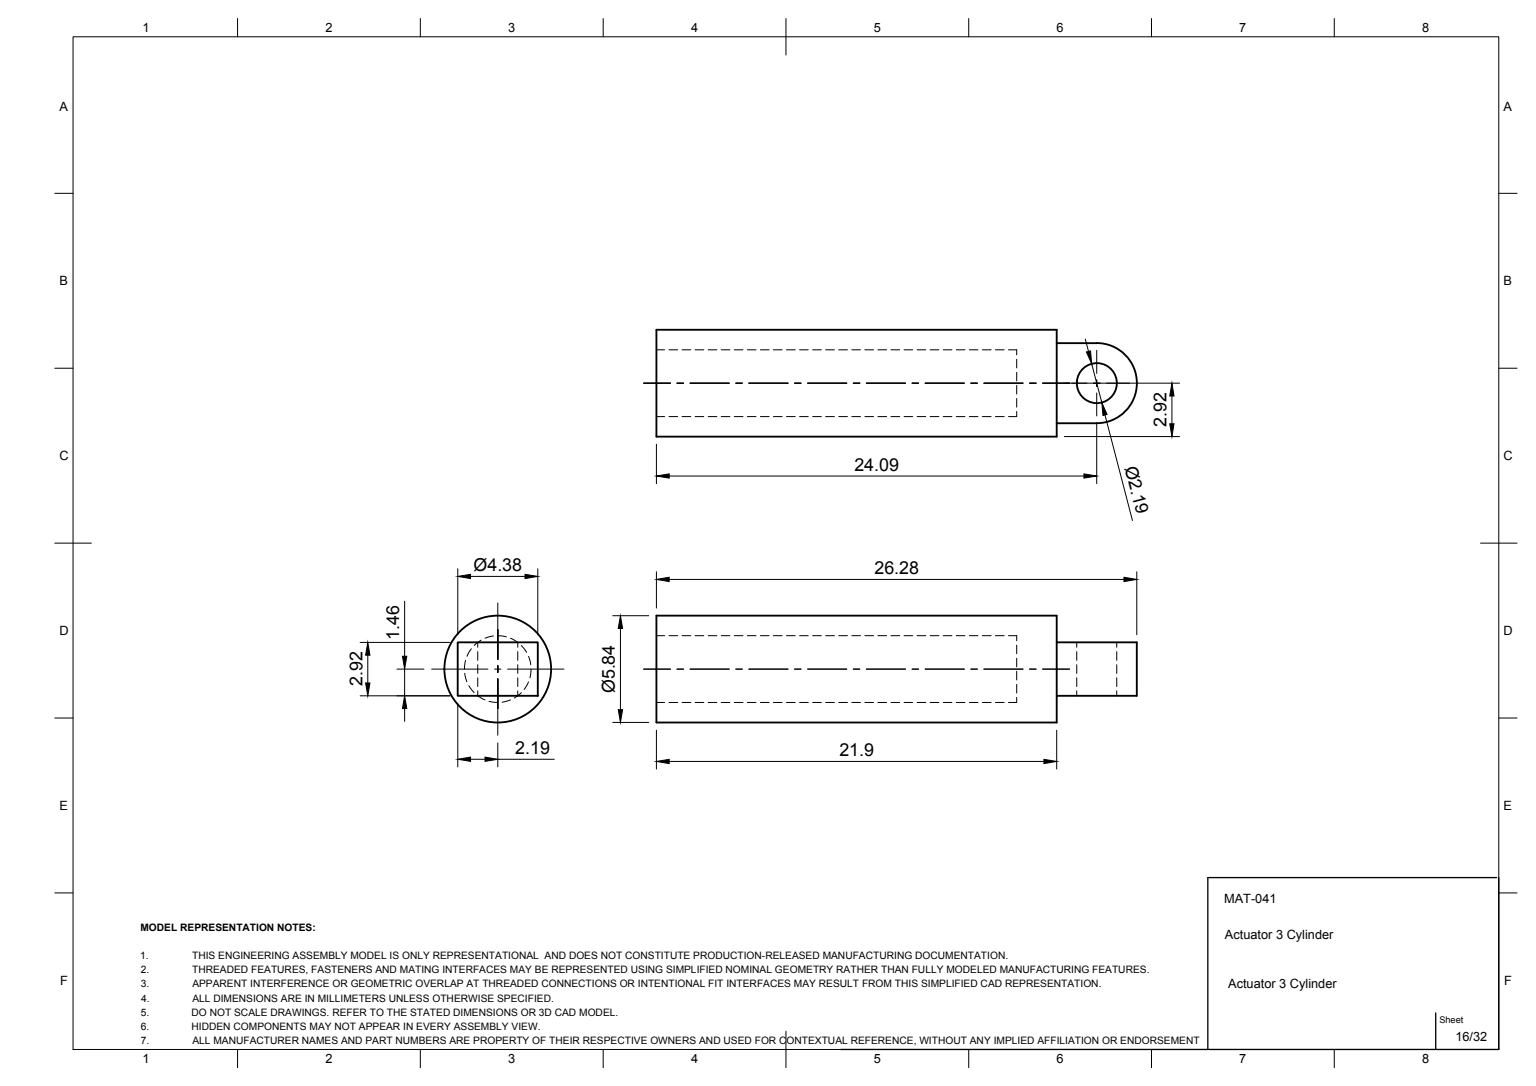
ISO-10303-21;
HEADER;
/* Generated by software containing ST-Developer
 * from STEP Tools, Inc. (www.steptools.com) 
 */

FILE_DESCRIPTION(
/* description */ ('STEP AP214'),
/* implementation_level */ '2;1');

FILE_NAME(
/* name */ 'Actuator 3 Cylinder.step',
/* time_stamp */ '2026-11-14T21:57:47-08:00',
/* author */ (''),
/* organization */ (''),
/* preprocessor_version */ 'ST-DEVELOPER v20.2',
/* originating_system */ 'Autodesk Translation Framework v15.17.0.0',
/* authorisation */ '');

FILE_SCHEMA (('AUTOMOTIVE_DESIGN { 1 0 10303 214 3 1 1 }'));
ENDSEC;

DATA;
#10=MECHANICAL_DESIGN_GEOMETRIC_PRESENTATION_REPRESENTATION('',(#254),#13199);
#218=SHAPE_REPRESENTATION_RELATIONSHIP('SRR','None',#13288,#236);
#236=ADVANCED_BREP_SHAPE_REPRESENTATION('',(#272),#13184);
#254=STYLED_ITEM('',(#13410),#272);
#272=MANIFOLD_SOLID_BREP('Body1',#6849);
#331=FACE_BOUND('',#2460,.T.);
#332=FACE_BOUND('',#2462,.T.);
#333=FACE_BOUND('',#2464,.T.);
#334=FACE_BOUND('',#2467,.T.);
#498=PLANE('',#7503);
#499=PLANE('',#7504);
#500=PLANE('',#7505);
#501=PLANE('',#7507);
#502=PLANE('',#7508);
#503=PLANE('',#7510);
#504=PLANE('',#7512);
#885=LINE('',#11682,#1403);
#886=LINE('',#11688,#1404);
#887=LINE('',#11694,#1405);
#888=LINE('',#11699,#1406);
#889=LINE('',#11701,#1407);
#890=LINE('',#11703,#1408);
#891=LINE('',#11704,#1409);
#892=LINE('',#11710,#1410);
#893=LINE('',#11711,#1411);
#894=LINE('',#11714,#1412);
#895=LINE('',#11715,#1413);
#896=LINE('',#11718,#1414);
#897=LINE('',#11721,#1415);
#1403=VECTOR('',#8976,1.825);
#1404=VECTOR('',#8983,1.095);
#1405=VECTOR('',#8990,2.92);
#1406=VECTOR('',#8995,1000.);
#1407=VECTOR('',#8996,1000.);
#1408=VECTOR('',#8997,1000.);
#1409=VECTOR('',#8998,1000.);
#1410=VECTOR('',#9005,1000.);
#1411=VECTOR('',#9006,1000.);
#1412=VECTOR('',#9009,1000.);
#1413=VECTOR('',#9010,1000.);
#1414=VECTOR('',#9013,1000.);
#1415=VECTOR('',#9018,1000.);
#1737=CYLINDRICAL_SURFACE('',#7494,1.825);
#1738=CYLINDRICAL_SURFACE('',#7497,1.095);
#1739=CYLINDRICAL_SURFACE('',#7500,2.92);
#1740=CYLINDRICAL_SURFACE('',#7511,2.19);
#2018=FACE_OUTER_BOUND('',#2456,.T.);
#2019=FACE_OUTER_BOUND('',#2457,.T.);
#2020=FACE_OUTER_BOUND('',#2458,.T.);
#2021=FACE_OUTER_BOUND('',#2459,.T.);
#2022=FACE_OUTER_BOUND('',#2461,.T.);
#2023=FACE_OUTER_BOUND('',#2463,.T.);
#2024=FACE_OUTER_BOUND('',#2465,.T.);
#2025=FACE_OUTER_BOUND('',#2466,.T.);
#2026=FACE_OUTER_BOUND('',#2468,.T.);
#2027=FACE_OUTER_BOUND('',#2469,.T.);
#2028=FACE_OUTER_BOUND('',#2470,.T.);
#2456=EDGE_LOOP('',(#5628,#5629,#5630,#5631));
#2457=EDGE_LOOP('',(#5632,#5633,#5634,#5635));
#2458=EDGE_LOOP('',(#5636,#5637,#5638,#5639));
#2459=EDGE_LOOP('',(#5640));
#2460=EDGE_LOOP('',(#5641,#5642,#5643,#5644));
#2461=EDGE_LOOP('',(#5645));
#2462=EDGE_LOOP('',(#5646));
#2463=EDGE_LOOP('',(#5647,#5648,#5649,#5650));
#2464=EDGE_LOOP('',(#5651));
#2465=EDGE_LOOP('',(#5652,#5653,#5654,#5655));
#2466=EDGE_LOOP('',(#5656,#5657,#5658,#5659));
#2467=EDGE_LOOP('',(#5660));
#2468=EDGE_LOOP('',(#5661,#5662,#5663,#5664));
#2469=EDGE_LOOP('',(#5665,#5666,#5667,#5668));
#2470=EDGE_LOOP('',(#5669));
#2875=CIRCLE('',#7495,1.825);
#2876=CIRCLE('',#7496,1.825);
#2877=CIRCLE('',#7498,1.095);
#2878=CIRCLE('',#7499,1.095);
#2879=CIRCLE('',#7501,2.92);
#2880=CIRCLE('',#7502,2.92);
#2881=CIRCLE('',#7506,2.19);
#2882=CIRCLE('',#7509,2.19);
#3344=VERTEX_POINT('',#11679);
#3345=VERTEX_POINT('',#11681);
#3346=VERTEX_POINT('',#11685);
#3347=VERTEX_POINT('',#11687);
#3348=VERTEX_POINT('',#11691);
#3349=VERTEX_POINT('',#11693);
#3350=VERTEX_POINT('',#11697);
#3351=VERTEX_POINT('',#11698);
#3352=VERTEX_POINT('',#11700);
#3353=VERTEX_POINT('',#11702);
#3354=VERTEX_POINT('',#11707);
#3355=VERTEX_POINT('',#11708);
#3356=VERTEX_POINT('',#11713);
#3357=VERTEX_POINT('',#11717);
#4151=EDGE_CURVE('',#3344,#3344,#2875,.T.);
#4152=EDGE_CURVE('',#3344,#3345,#885,.T.);
#4153=EDGE_CURVE('',#3345,#3345,#2876,.T.);
#4154=EDGE_CURVE('',#3346,#3346,#2877,.T.);
#4155=EDGE_CURVE('',#3346,#3347,#886,.T.);
#4156=EDGE_CURVE('',#3347,#3347,#2878,.T.);
#4157=EDGE_CURVE('',#3348,#3348,#2879,.T.);
#4158=EDGE_CURVE('',#3348,#3349,#887,.T.);
#4159=EDGE_CURVE('',#3349,#3349,#2880,.T.);
#4160=EDGE_CURVE('',#3350,#3351,#888,.T.);
#4161=EDGE_CURVE('',#3352,#3350,#889,.T.);
#4162=EDGE_CURVE('',#3353,#3352,#890,.T.);
#4163=EDGE_CURVE('',#3351,#3353,#891,.T.);
#4164=EDGE_CURVE('',#3354,#3355,#2881,.T.);
#4165=EDGE_CURVE('',#3355,#3350,#892,.T.);
#4166=EDGE_CURVE('',#3354,#3351,#893,.T.);
#4167=EDGE_CURVE('',#3356,#3353,#894,.T.);
#4168=EDGE_CURVE('',#3356,#3354,#895,.T.);
#4169=EDGE_CURVE('',#3357,#3352,#896,.T.);
#4170=EDGE_CURVE('',#3357,#3356,#2882,.T.);
#4171=EDGE_CURVE('',#3355,#3357,#897,.T.);
#5628=ORIENTED_EDGE('',*,*,#4151,.F.);
#5629=ORIENTED_EDGE('',*,*,#4152,.T.);
#5630=ORIENTED_EDGE('',*,*,#4153,.T.);
#5631=ORIENTED_EDGE('',*,*,#4152,.F.);
#5632=ORIENTED_EDGE('',*,*,#4154,.F.);
#5633=ORIENTED_EDGE('',*,*,#4155,.T.);
#5634=ORIENTED_EDGE('',*,*,#4156,.T.);
#5635=ORIENTED_EDGE('',*,*,#4155,.F.);
#5636=ORIENTED_EDGE('',*,*,#4157,.T.);
#5637=ORIENTED_EDGE('',*,*,#4158,.T.);
#5638=ORIENTED_EDGE('',*,*,#4159,.F.);
#5639=ORIENTED_EDGE('',*,*,#4158,.F.);
#5640=ORIENTED_EDGE('',*,*,#4157,.F.);
#5641=ORIENTED_EDGE('',*,*,#4160,.F.);
#5642=ORIENTED_EDGE('',*,*,#4161,.F.);
#5643=ORIENTED_EDGE('',*,*,#4162,.F.);
#5644=ORIENTED_EDGE('',*,*,#4163,.F.);
#5645=ORIENTED_EDGE('',*,*,#4159,.T.);
#5646=ORIENTED_EDGE('',*,*,#4153,.F.);
#5647=ORIENTED_EDGE('',*,*,#4164,.T.);
#5648=ORIENTED_EDGE('',*,*,#4165,.T.);
#5649=ORIENTED_EDGE('',*,*,#4160,.T.);
#5650=ORIENTED_EDGE('',*,*,#4166,.F.);
#5651=ORIENTED_EDGE('',*,*,#4154,.T.);
#5652=ORIENTED_EDGE('',*,*,#4167,.F.);
#5653=ORIENTED_EDGE('',*,*,#4168,.T.);
#5654=ORIENTED_EDGE('',*,*,#4166,.T.);
#5655=ORIENTED_EDGE('',*,*,#4163,.T.);
#5656=ORIENTED_EDGE('',*,*,#4169,.F.);
#5657=ORIENTED_EDGE('',*,*,#4170,.T.);
#5658=ORIENTED_EDGE('',*,*,#4167,.T.);
#5659=ORIENTED_EDGE('',*,*,#4162,.T.);
#5660=ORIENTED_EDGE('',*,*,#4156,.F.);
#5661=ORIENTED_EDGE('',*,*,#4165,.F.);
#5662=ORIENTED_EDGE('',*,*,#4171,.T.);
#5663=ORIENTED_EDGE('',*,*,#4169,.T.);
#5664=ORIENTED_EDGE('',*,*,#4161,.T.);
#5665=ORIENTED_EDGE('',*,*,#4168,.F.);
#5666=ORIENTED_EDGE('',*,*,#4170,.F.);
#5667=ORIENTED_EDGE('',*,*,#4171,.F.);
#5668=ORIENTED_EDGE('',*,*,#4164,.F.);
#5669=ORIENTED_EDGE('',*,*,#4151,.T.);
#6670=ADVANCED_FACE('',(#2018),#1737,.F.);
#6671=ADVANCED_FACE('',(#2019),#1738,.F.);
#6672=ADVANCED_FACE('',(#2020),#1739,.T.);
#6673=ADVANCED_FACE('',(#2021,#331),#498,.F.);
#6674=ADVANCED_FACE('',(#2022,#332),#499,.T.);
#6675=ADVANCED_FACE('',(#2023,#333),#500,.F.);
#6676=ADVANCED_FACE('',(#2024),#501,.F.);
#6677=ADVANCED_FACE('',(#2025,#334),#502,.F.);
#6678=ADVANCED_FACE('',(#2026),#503,.F.);
#6679=ADVANCED_FACE('',(#2027),#1740,.T.);
#6680=ADVANCED_FACE('',(#2028),#504,.T.);
#6849=CLOSED_SHELL('',(#6670,#6671,#6672,#6673,#6674,#6675,#6676,#6677,
#6678,#6679,#6680));
#7493=AXIS2_PLACEMENT_3D('',#11677,#8970,#8971);
#7494=AXIS2_PLACEMENT_3D('',#11678,#8972,#8973);
#7495=AXIS2_PLACEMENT_3D('',#11680,#8974,#8975);
#7496=AXIS2_PLACEMENT_3D('',#11683,#8977,#8978);
#7497=AXIS2_PLACEMENT_3D('',#11684,#8979,#8980);
#7498=AXIS2_PLACEMENT_3D('',#11686,#8981,#8982);
#7499=AXIS2_PLACEMENT_3D('',#11689,#8984,#8985);
#7500=AXIS2_PLACEMENT_3D('',#11690,#8986,#8987);
#7501=AXIS2_PLACEMENT_3D('',#11692,#8988,#8989);
#7502=AXIS2_PLACEMENT_3D('',#11695,#8991,#8992);
#7503=AXIS2_PLACEMENT_3D('',#11696,#8993,#8994);
#7504=AXIS2_PLACEMENT_3D('',#11705,#8999,#9000);
#7505=AXIS2_PLACEMENT_3D('',#11706,#9001,#9002);
#7506=AXIS2_PLACEMENT_3D('',#11709,#9003,#9004);
#7507=AXIS2_PLACEMENT_3D('',#11712,#9007,#9008);
#7508=AXIS2_PLACEMENT_3D('',#11716,#9011,#9012);
#7509=AXIS2_PLACEMENT_3D('',#11719,#9014,#9015);
#7510=AXIS2_PLACEMENT_3D('',#11720,#9016,#9017);
#7511=AXIS2_PLACEMENT_3D('',#11722,#9019,#9020);
#7512=AXIS2_PLACEMENT_3D('',#11723,#9021,#9022);
#8970=DIRECTION('axis',(0.,0.,1.));
#8971=DIRECTION('refdir',(1.,0.,0.));
#8972=DIRECTION('center_axis',(0.,0.,1.));
#8973=DIRECTION('ref_axis',(1.,0.,0.));
#8974=DIRECTION('center_axis',(0.,0.,1.));
#8975=DIRECTION('ref_axis',(1.,0.,0.));
#8976=DIRECTION('',(0.,0.,1.));
#8977=DIRECTION('center_axis',(0.,0.,1.));
#8978=DIRECTION('ref_axis',(1.,0.,0.));
#8979=DIRECTION('center_axis',(1.,-1.0842021724855E-16,0.));
#8980=DIRECTION('ref_axis',(1.0842021724855E-16,1.,0.));
#8981=DIRECTION('center_axis',(1.,-7.2280144832367E-17,0.));
#8982=DIRECTION('ref_axis',(7.2280144832367E-17,1.,0.));
#8983=DIRECTION('',(1.,-1.0842021724855E-16,0.));
#8984=DIRECTION('center_axis',(1.,-1.0842021724855E-16,0.));
#8985=DIRECTION('ref_axis',(1.0842021724855E-16,1.,0.));
#8986=DIRECTION('center_axis',(0.,0.,-1.));
#8987=DIRECTION('ref_axis',(-1.,0.,0.));
#8988=DIRECTION('center_axis',(0.,0.,1.));
#8989=DIRECTION('ref_axis',(1.,0.,0.));
#8990=DIRECTION('',(0.,0.,1.));
#8991=DIRECTION('center_axis',(0.,0.,1.));
#8992=DIRECTION('ref_axis',(1.,0.,0.));
#8993=DIRECTION('center_axis',(0.,0.,1.));
#8994=DIRECTION('ref_axis',(1.,0.,0.));
#8995=DIRECTION('',(7.2280144832367E-17,1.,0.));
#8996=DIRECTION('',(-1.,0.,0.));
#8997=DIRECTION('',(-1.44560289664734E-16,-1.,0.));
#8998=DIRECTION('',(1.,0.,0.));
#8999=DIRECTION('center_axis',(0.,0.,1.));
#9000=DIRECTION('ref_axis',(1.,0.,0.));
#9001=DIRECTION('center_axis',(1.,-7.2280144832367E-17,0.));
#9002=DIRECTION('ref_axis',(7.2280144832367E-17,1.,0.));
#9003=DIRECTION('center_axis',(-1.,7.2280144832367E-17,0.));
#9004=DIRECTION('ref_axis',(7.2280144832367E-17,1.,0.));
#9005=DIRECTION('',(0.,0.,1.));
#9006=DIRECTION('',(0.,0.,1.));
#9007=DIRECTION('center_axis',(0.,-1.,0.));
#9008=DIRECTION('ref_axis',(0.,0.,-1.));
#9009=DIRECTION('',(0.,0.,1.));
#9010=DIRECTION('',(-1.,0.,0.));
#9011=DIRECTION('center_axis',(-1.,1.44560289664734E-16,0.));
#9012=DIRECTION('ref_axis',(-1.44560289664734E-16,-1.,0.));
#9013=DIRECTION('',(0.,0.,1.));
#9014=DIRECTION('center_axis',(1.,-1.44560289664734E-16,0.));
#9015=DIRECTION('ref_axis',(-1.44560289664734E-16,-1.,0.));
#9016=DIRECTION('center_axis',(0.,1.,0.));
#9017=DIRECTION('ref_axis',(0.,0.,1.));
#9018=DIRECTION('',(1.,0.,0.));
#9019=DIRECTION('center_axis',(-1.,0.,0.));
#9020=DIRECTION('ref_axis',(0.,1.22464679914735E-16,-1.));
#9021=DIRECTION('center_axis',(0.,0.,1.));
#9022=DIRECTION('ref_axis',(1.,0.,0.));
#11677=CARTESIAN_POINT('',(0.,0.,0.));
#11678=CARTESIAN_POINT('Origin',(6.03700957585037E-17,-6.47376725810661E-18,
5.59782889707835));
#11679=CARTESIAN_POINT('',(-1.825,-2.29971808102499E-16,5.59782889707835));
#11680=CARTESIAN_POINT('Origin',(6.03700957585037E-17,-6.47376725810661E-18,
5.59782889707835));
#11681=CARTESIAN_POINT('',(-1.825,-2.29971808102499E-16,25.3078288970784));
#11682=CARTESIAN_POINT('',(-1.825,-2.29971808102499E-16,5.59782889707835));
#11683=CARTESIAN_POINT('Origin',(6.03700957585037E-17,-6.47376725810661E-18,
25.3078288970784));
#11684=CARTESIAN_POINT('Origin',(-2.92,3.76068899267196E-16,1.21782889707835));
#11685=CARTESIAN_POINT('',(-1.46,-1.095,1.21782889707835));
#11686=CARTESIAN_POINT('Origin',(-1.46,2.17775382084312E-16,1.21782889707835));
#11687=CARTESIAN_POINT('',(1.46,-1.095,1.21782889707835));
#11688=CARTESIAN_POINT('',(-2.92,-1.095,1.21782889707835));
#11689=CARTESIAN_POINT('Origin',(1.46,-9.88116522814554E-17,1.21782889707835));
#11690=CARTESIAN_POINT('Origin',(6.03700957585037E-17,-6.47376725810661E-18,
25.3078288970784));
#11691=CARTESIAN_POINT('',(2.92,-3.64070632609134E-16,3.40782889707835));
#11692=CARTESIAN_POINT('Origin',(6.03700957585037E-17,-6.47376725810661E-18,
3.40782889707835));
#11693=CARTESIAN_POINT('',(2.92,-3.64070632609134E-16,25.3078288970784));
#11694=CARTESIAN_POINT('',(2.92,-3.64070632609134E-16,25.3078288970784));
#11695=CARTESIAN_POINT('Origin',(6.03700957585037E-17,-6.47376725810661E-18,
25.3078288970784));
#11696=CARTESIAN_POINT('Origin',(6.03700957585037E-17,-6.47376725810661E-18,
3.40782889707835));
#11697=CARTESIAN_POINT('',(-1.46,-2.19,3.40782889707835));
#11698=CARTESIAN_POINT('',(-1.46,2.19,3.40782889707835));
#11699=CARTESIAN_POINT('',(-1.46,2.19,3.40782889707835));
#11700=CARTESIAN_POINT('',(1.46,-2.19,3.40782889707835));
#11701=CARTESIAN_POINT('',(1.46,-2.19,3.40782889707835));
#11702=CARTESIAN_POINT('',(1.46,2.19,3.40782889707835));
#11703=CARTESIAN_POINT('',(1.46,2.19,3.40782889707835));
#11704=CARTESIAN_POINT('',(1.46,2.19,3.40782889707835));
#11705=CARTESIAN_POINT('Origin',(6.03700957585037E-17,-6.47376725810661E-18,
25.3078288970784));
#11706=CARTESIAN_POINT('Origin',(-1.46,2.19,-0.972171102921649));
#11707=CARTESIAN_POINT('',(-1.46,2.19,1.21782889707835));
#11708=CARTESIAN_POINT('',(-1.46,-2.19,1.21782889707835));
#11709=CARTESIAN_POINT('Origin',(-1.46,-6.47376725810661E-18,1.21782889707835));
#11710=CARTESIAN_POINT('',(-1.46,-2.19,-0.972171102921649));
#11711=CARTESIAN_POINT('',(-1.46,2.19,-0.972171102921649));
#11712=CARTESIAN_POINT('Origin',(1.46,2.19,-0.972171102921649));
#11713=CARTESIAN_POINT('',(1.46,2.19,1.21782889707835));
#11714=CARTESIAN_POINT('',(1.46,2.19,-0.972171102921649));
#11715=CARTESIAN_POINT('',(-1.46,2.19,1.21782889707835));
#11716=CARTESIAN_POINT('Origin',(1.46,2.19,-0.972171102921649));
#11717=CARTESIAN_POINT('',(1.46,-2.19,1.21782889707835));
#11718=CARTESIAN_POINT('',(1.46,-2.19,-0.972171102921649));
#11719=CARTESIAN_POINT('Origin',(1.46,-6.47376725810661E-18,1.21782889707835));
#11720=CARTESIAN_POINT('Origin',(1.46,-2.19,-0.972171102921649));
#11721=CARTESIAN_POINT('',(1.46,-2.19,1.21782889707835));
#11722=CARTESIAN_POINT('Origin',(6.03700957585037E-17,-6.47376725810661E-18,
1.21782889707835));
#11723=CARTESIAN_POINT('Origin',(6.03700957585037E-17,-6.47376725810661E-18,
5.59782889707835));
#13158=UNCERTAINTY_MEASURE_WITH_UNIT(LENGTH_MEASURE(0.01),#13200,
'DISTANCE_ACCURACY_VALUE',
'Maximum model space distance between geometric entities at asserted c
onnectivities');
#13173=UNCERTAINTY_MEASURE_WITH_UNIT(LENGTH_MEASURE(0.01),#13200,
'DISTANCE_ACCURACY_VALUE',
'Maximum model space distance between geometric entities at asserted c
onnectivities');
#13184=(
GEOMETRIC_REPRESENTATION_CONTEXT(3)
GLOBAL_UNCERTAINTY_ASSIGNED_CONTEXT((#13158))
GLOBAL_UNIT_ASSIGNED_CONTEXT((#13200,#13202,#13203))
REPRESENTATION_CONTEXT('','3D')
);
#13199=(
GEOMETRIC_REPRESENTATION_CONTEXT(3)
GLOBAL_UNCERTAINTY_ASSIGNED_CONTEXT((#13173))
GLOBAL_UNIT_ASSIGNED_CONTEXT((#13200,#13202,#13203))
REPRESENTATION_CONTEXT('','3D')
);
#13200=(
LENGTH_UNIT()
NAMED_UNIT(*)
SI_UNIT(.MILLI.,.METRE.)
);
#13202=(
NAMED_UNIT(*)
PLANE_ANGLE_UNIT()
SI_UNIT($,.RADIAN.)
);
#13203=(
NAMED_UNIT(*)
SI_UNIT($,.STERADIAN.)
SOLID_ANGLE_UNIT()
);
#13214=SHAPE_DEFINITION_REPRESENTATION(#13241,#13288);
#13241=PRODUCT_DEFINITION_SHAPE('',$,#13314);
#13288=SHAPE_REPRESENTATION('',(#7493),#13184);
#13303=PRODUCT_DEFINITION_CONTEXT('part definition',#13380,'design');
#13314=PRODUCT_DEFINITION('Actuator 3 Cylinder','Actuator 3 Cylinder',#13339,
#13303);
#13339=PRODUCT_DEFINITION_FORMATION('',$,#13392);
#13380=APPLICATION_CONTEXT(
'Core Data for Automotive Mechanical Design Process');
#13381=PRODUCT_CONTEXT('part definition',#13380,'mechanical');
#13392=PRODUCT('Actuator 3 Cylinder','Actuator 3 Cylinder',$,(#13381));
#13410=PRESENTATION_STYLE_ASSIGNMENT((#13415));
#13415=SURFACE_STYLE_USAGE(.BOTH.,#13420);
#13420=SURFACE_SIDE_STYLE('',(#13425));
#13425=SURFACE_STYLE_FILL_AREA(#13430);
#13430=FILL_AREA_STYLE('Opaque(227,224,212)',(#13435));
#13435=FILL_AREA_STYLE_COLOUR('Opaque(227,224,212)',#13440);
#13440=COLOUR_RGB('Opaque(227,224,212)',0.890196078431372,0.87843137254902,
0.831372549019608);
ENDSEC;
END-ISO-10303-21;
